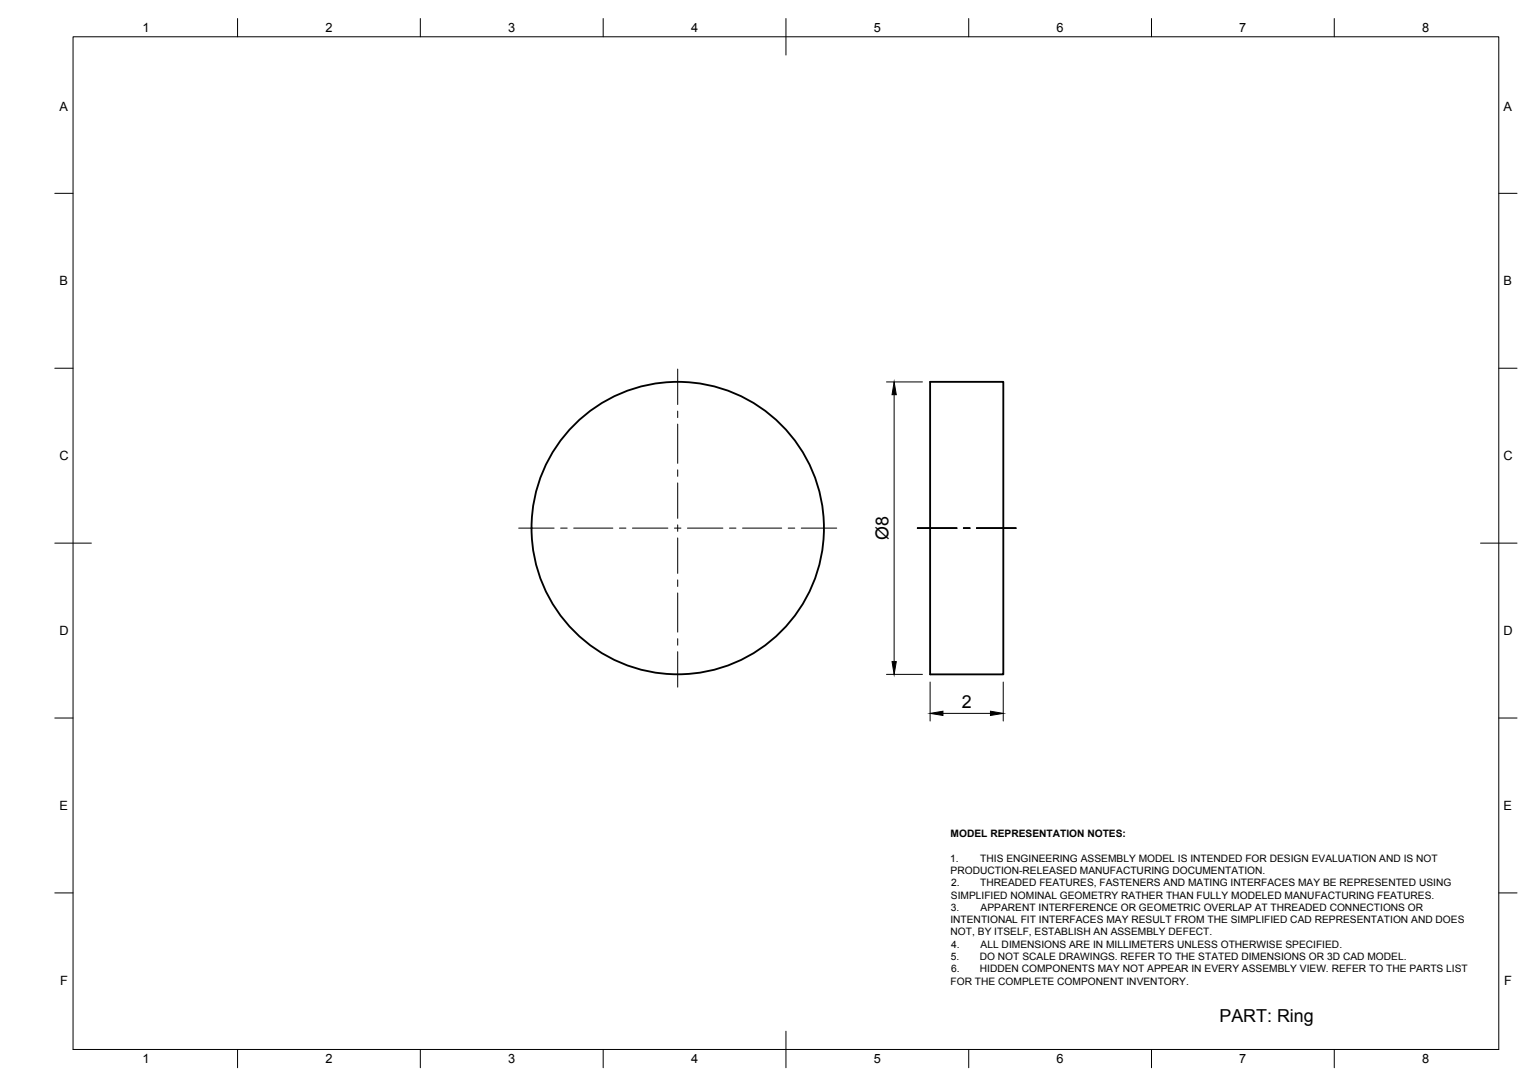
ISO-10303-21;
HEADER;
/* Generated by software containing ST-Developer
 * from STEP Tools, Inc. (www.steptools.com) 
 */

FILE_DESCRIPTION(
/* description */ (''),
/* implementation_level */ '2;1');

FILE_NAME(
/* name */ 'Ring.step',
/* time_stamp */ '2026-10-05T01:33:24-07:00',
/* author */ (''),
/* organization */ (''),
/* preprocessor_version */ 'ST-DEVELOPER v20.2',
/* originating_system */ 'Autodesk Translation Framework v15.15.0.0',
/* authorisation */ '');

FILE_SCHEMA (('AUTOMOTIVE_DESIGN { 1 0 10303 214 3 1 1 }'));
ENDSEC;

DATA;
#10=MECHANICAL_DESIGN_GEOMETRIC_PRESENTATION_REPRESENTATION('',(#87),#1128);
#67=SHAPE_REPRESENTATION_RELATIONSHIP('SRR','None',#1171,#77);
#77=ADVANCED_BREP_SHAPE_REPRESENTATION('',(#97),#1123);
#87=STYLED_ITEM('',(#1227),#97);
#97=MANIFOLD_SOLID_BREP('Body1',#526);
#110=LINE('',#1034,#127);
#127=VECTOR('',#853,4.);
#141=CYLINDRICAL_SURFACE('',#693,4.);
#167=FACE_OUTER_BOUND('',#208,.T.);
#168=FACE_OUTER_BOUND('',#209,.T.);
#169=FACE_OUTER_BOUND('',#210,.T.);
#208=EDGE_LOOP('',(#406));
#209=EDGE_LOOP('',(#407));
#210=EDGE_LOOP('',(#408,#409,#410,#411));
#247=CIRCLE('',#690,4.);
#248=CIRCLE('',#692,4.);
#281=VERTEX_POINT('',#1028);
#282=VERTEX_POINT('',#1031);
#325=EDGE_CURVE('',#281,#281,#247,.T.);
#326=EDGE_CURVE('',#282,#282,#248,.T.);
#327=EDGE_CURVE('',#281,#282,#110,.T.);
#406=ORIENTED_EDGE('',*,*,#325,.T.);
#407=ORIENTED_EDGE('',*,*,#326,.F.);
#408=ORIENTED_EDGE('',*,*,#325,.F.);
#409=ORIENTED_EDGE('',*,*,#327,.T.);
#410=ORIENTED_EDGE('',*,*,#326,.T.);
#411=ORIENTED_EDGE('',*,*,#327,.F.);
#470=PLANE('',#689);
#471=PLANE('',#691);
#501=ADVANCED_FACE('',(#167),#470,.T.);
#502=ADVANCED_FACE('',(#168),#471,.T.);
#503=ADVANCED_FACE('',(#169),#141,.T.);
#526=CLOSED_SHELL('',(#501,#502,#503));
#688=AXIS2_PLACEMENT_3D('',#1026,#841,#842);
#689=AXIS2_PLACEMENT_3D('',#1027,#843,#844);
#690=AXIS2_PLACEMENT_3D('',#1029,#845,#846);
#691=AXIS2_PLACEMENT_3D('',#1030,#847,#848);
#692=AXIS2_PLACEMENT_3D('',#1032,#849,#850);
#693=AXIS2_PLACEMENT_3D('',#1033,#851,#852);
#841=DIRECTION('axis',(0.,0.,1.));
#842=DIRECTION('refdir',(1.,0.,0.));
#843=DIRECTION('center_axis',(1.,0.,0.));
#844=DIRECTION('ref_axis',(0.,0.,-1.));
#845=DIRECTION('center_axis',(1.,0.,0.));
#846=DIRECTION('ref_axis',(0.,0.,-1.));
#847=DIRECTION('center_axis',(-1.,0.,0.));
#848=DIRECTION('ref_axis',(0.,0.,1.));
#849=DIRECTION('center_axis',(1.,0.,0.));
#850=DIRECTION('ref_axis',(0.,0.,-1.));
#851=DIRECTION('center_axis',(1.,0.,0.));
#852=DIRECTION('ref_axis',(0.,0.,-1.));
#853=DIRECTION('',(-1.,0.,0.));
#1026=CARTESIAN_POINT('',(0.,0.,0.));
#1027=CARTESIAN_POINT('Origin',(20.2354431734887,0.,0.));
#1028=CARTESIAN_POINT('',(20.2354431734887,-4.89858719658941E-16,4.));
#1029=CARTESIAN_POINT('Origin',(20.2354431734887,0.,0.));
#1030=CARTESIAN_POINT('Origin',(18.2354431734887,0.,-4.));
#1031=CARTESIAN_POINT('',(18.2354431734887,-4.89858719658941E-16,4.));
#1032=CARTESIAN_POINT('Origin',(18.2354431734887,0.,0.));
#1033=CARTESIAN_POINT('Origin',(19.2354431734887,0.,0.));
#1034=CARTESIAN_POINT('',(19.2354431734887,-4.89858719658941E-16,4.));
#1111=UNCERTAINTY_MEASURE_WITH_UNIT(LENGTH_MEASURE(0.01),#1129,
'DISTANCE_ACCURACY_VALUE',
'Maximum model space distance between geometric entities at asserted c
onnectivities');
#1116=UNCERTAINTY_MEASURE_WITH_UNIT(LENGTH_MEASURE(0.01),#1129,
'DISTANCE_ACCURACY_VALUE',
'Maximum model space distance between geometric entities at asserted c
onnectivities');
#1123=(
GEOMETRIC_REPRESENTATION_CONTEXT(3)
GLOBAL_UNCERTAINTY_ASSIGNED_CONTEXT((#1111))
GLOBAL_UNIT_ASSIGNED_CONTEXT((#1129,#1131,#1132))
REPRESENTATION_CONTEXT('','3D')
);
#1128=(
GEOMETRIC_REPRESENTATION_CONTEXT(3)
GLOBAL_UNCERTAINTY_ASSIGNED_CONTEXT((#1116))
GLOBAL_UNIT_ASSIGNED_CONTEXT((#1129,#1131,#1132))
REPRESENTATION_CONTEXT('','3D')
);
#1129=(
LENGTH_UNIT()
NAMED_UNIT(*)
SI_UNIT(.MILLI.,.METRE.)
);
#1131=(
NAMED_UNIT(*)
PLANE_ANGLE_UNIT()
SI_UNIT($,.RADIAN.)
);
#1132=(
NAMED_UNIT(*)
SI_UNIT($,.STERADIAN.)
SOLID_ANGLE_UNIT()
);
#1139=SHAPE_DEFINITION_REPRESENTATION(#1150,#1171);
#1150=PRODUCT_DEFINITION_SHAPE('',$,#1183);
#1171=SHAPE_REPRESENTATION('',(#688),#1123);
#1176=PRODUCT_DEFINITION_CONTEXT('part definition',#1211,'design');
#1183=PRODUCT_DEFINITION('Ring','Ring',#1194,#1176);
#1194=PRODUCT_DEFINITION_FORMATION('',$,#1219);
#1211=APPLICATION_CONTEXT(
'Core Data for Automotive Mechanical Design Process');
#1212=PRODUCT_CONTEXT('part definition',#1211,'mechanical');
#1219=PRODUCT('Ring','Ring',$,(#1212));
#1227=PRESENTATION_STYLE_ASSIGNMENT((#1231));
#1231=SURFACE_STYLE_USAGE(.BOTH.,#1235);
#1235=SURFACE_SIDE_STYLE('',(#1239));
#1239=SURFACE_STYLE_FILL_AREA(#1243);
#1243=FILL_AREA_STYLE('Opaque(77,77,77)',(#1247));
#1247=FILL_AREA_STYLE_COLOUR('Opaque(77,77,77)',#1251);
#1251=COLOUR_RGB('Opaque(77,77,77)', 0.72549020, 0.75294118, 0.79215686);
ENDSEC;
END-ISO-10303-21;
